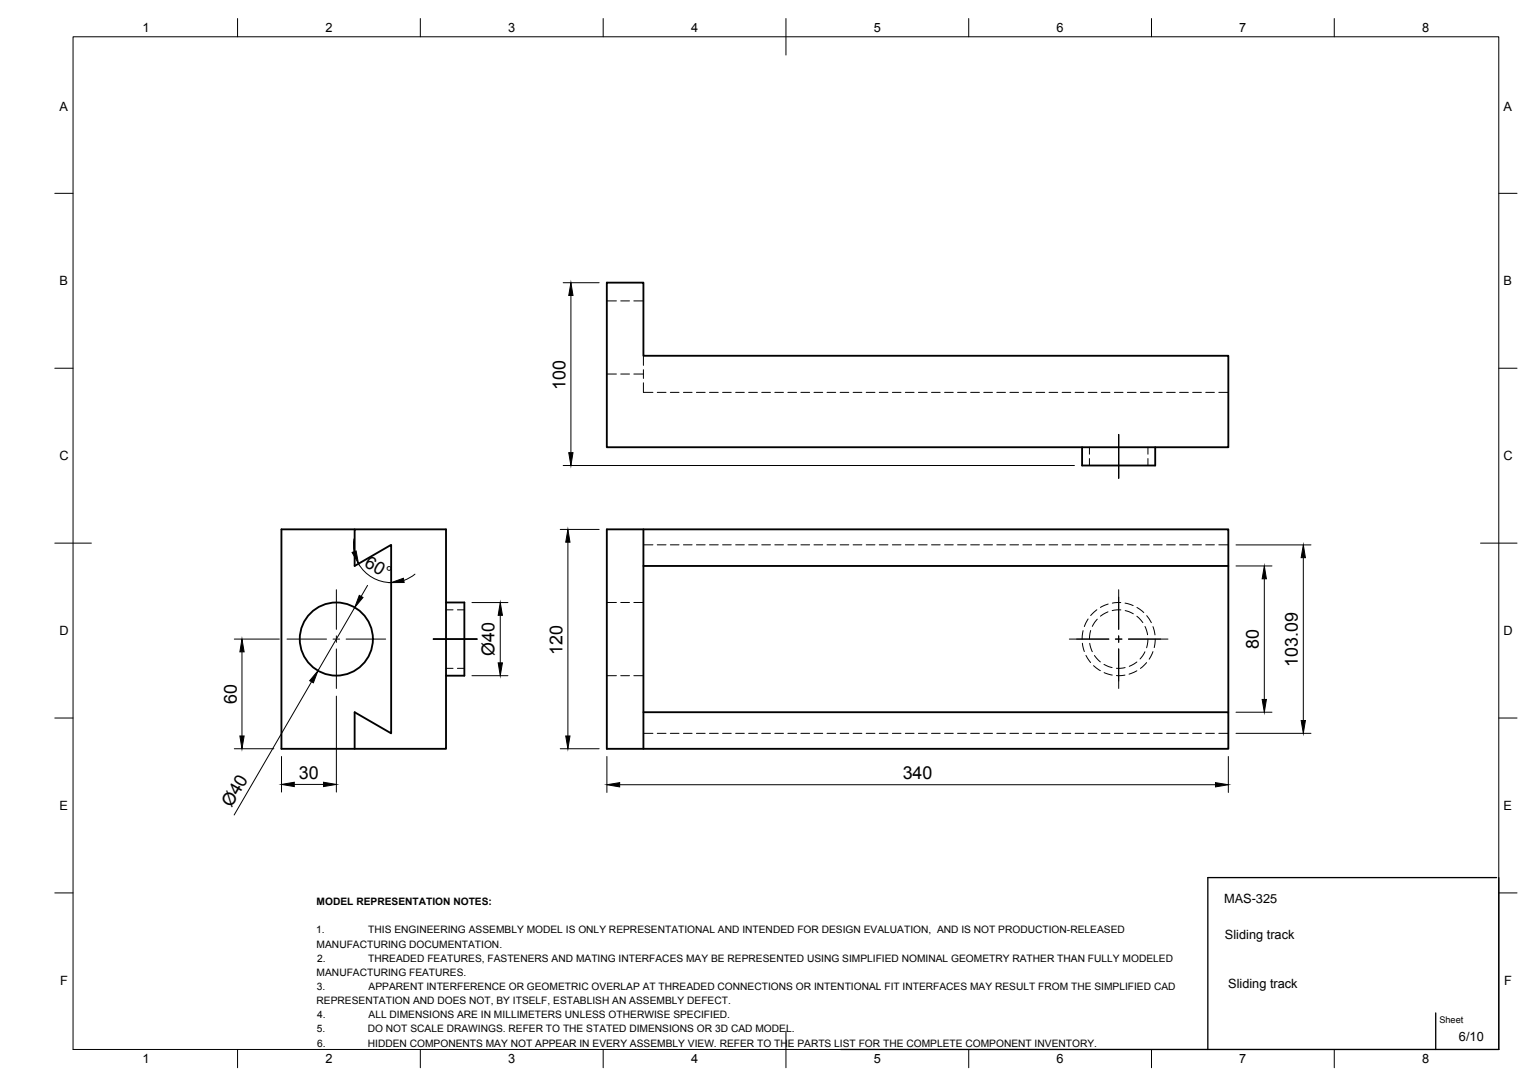
ISO-10303-21;
HEADER;
FILE_DESCRIPTION (('STEP AP214'),
    '1' );
FILE_NAME ('Sliding track.step',
    '2026-10-08T01:23:29',
    ( '' ),
    ( '' ),
    'SwSTEP 2.0',
    'SolidWorks 2025',
    '' );
FILE_SCHEMA (( 'AUTOMOTIVE_DESIGN' ));
ENDSEC;

DATA;
#68=ORIENTED_EDGE ( 'NONE', *, *, #41329, .T. ) ;
#133=LINE ( 'NONE', #35615, #5709 ) ;
#139=EDGE_LOOP ( 'NONE', ( #49981, #10287, #23201, #19361 ) ) ;
#158=DIRECTION ( 'NONE',  ( 0.000000000000000000, 0.000000000000000000, 1.000000000000000000 ) ) ;
#254=CARTESIAN_POINT ( 'NONE',  ( 1.959434878635765131E-15, -63.50000000000000000, 16.00000000000000000 ) ) ;
#289=VECTOR ( 'NONE', #42767, 1000.000000000000000 ) ;
#296=ORIENTED_EDGE ( 'NONE', *, *, #7021, .F. ) ;
#314=CARTESIAN_POINT ( 'NONE',  ( 60.00000000000000000, -113.5000000000000000, 60.00000000000000711 ) ) ;
#367=ADVANCED_FACE ( 'NONE', ( #12542 ), #28557, .F. ) ;
#505=VECTOR ( 'NONE', #2539, 1000.000000000000000 ) ;
#580=DIRECTION ( 'NONE',  ( 0.000000000000000000, 0.000000000000000000, 1.000000000000000000 ) ) ;
#689=AXIS2_PLACEMENT_3D ( 'NONE', #43278, #30663, #18596 ) ;
#692=CARTESIAN_POINT ( 'NONE',  ( 60.00000000000000000, -113.5000000000000000, 60.00000000000000711 ) ) ;
#701=VECTOR ( 'NONE', #47280, 1000.000000000000000 ) ;
#766=ORIENTED_EDGE ( 'NONE', *, *, #47209, .F. ) ;
#828=CARTESIAN_POINT ( 'NONE',  ( -260.0000000000000000, -113.5000000000000000, -40.00000000000001421 ) ) ;
#915=VECTOR ( 'NONE', #37349, 1000.000000000000000 ) ;
#918=FACE_OUTER_BOUND ( 'NONE', #42235, .T. ) ;
#921=EDGE_CURVE ( 'NONE', #5941, #31777, #13986, .T. ) ;
#924=CARTESIAN_POINT ( 'NONE',  ( -260.0000000000000000, -113.5000000000000142, 60.00000000000001421 ) ) ;
#941=CARTESIAN_POINT ( 'NONE',  ( 0.000000000000000000, -53.50000000000000000, 0.000000000000000000 ) ) ;
#1043=PRODUCT_DEFINITION ( 'UNKNOWN', '', #41839, #39510 ) ;
#1058=AXIS2_PLACEMENT_3D ( 'NONE', #5694, #20664, #36698 ) ;
#1110=DIRECTION ( 'NONE',  ( 0.000000000000000000, 0.000000000000000000, -1.000000000000000000 ) ) ;
#1120=CARTESIAN_POINT ( 'NONE',  ( -280.0000000000000000, -63.50000000000000000, 60.00000000000000711 ) ) ;
#1155=DIRECTION ( 'NONE',  ( -0.000000000000000000, 1.156482317317871232E-16, 1.000000000000000000 ) ) ;
#1226=CARTESIAN_POINT ( 'NONE',  ( -260.0000000000000000, -113.5000000000000142, -60.00000000000001421 ) ) ;
#1229=FACE_BOUND ( 'NONE', #16915, .T. ) ;
#1237=ORIENTED_EDGE ( 'NONE', *, *, #23580, .T. ) ;
#1312=ORIENTED_EDGE ( 'NONE', *, *, #8264, .T. ) ;
#1383=CYLINDRICAL_SURFACE ( 'NONE', #44480, 20.00000000000000000 ) ;
#1444=DIRECTION ( 'NONE',  ( 1.000000000000000000, -0.000000000000000000, 0.000000000000000000 ) ) ;
#1544=LINE ( 'NONE', #13627, #43335 ) ;
#1696=CARTESIAN_POINT ( 'NONE',  ( 0.000000000000000000, -53.50000000000000000, 0.000000000000000000 ) ) ;
#1848=FACE_OUTER_BOUND ( 'NONE', #42521, .T. ) ;
#2052=DIRECTION ( 'NONE',  ( -0.000000000000000000, -1.000000000000000000, -0.000000000000000000 ) ) ;
#2064=VERTEX_POINT ( 'NONE', #8952 ) ;
#2160=ORIENTED_EDGE ( 'NONE', *, *, #11113, .T. ) ;
#2332=CARTESIAN_POINT ( 'NONE',  ( 0.000000000000000000, -53.50000000000000000, -16.00000000000000000 ) ) ;
#2380=( GEOMETRIC_REPRESENTATION_CONTEXT ( 3 ) GLOBAL_UNCERTAINTY_ASSIGNED_CONTEXT ( ( #14323 ) ) GLOBAL_UNIT_ASSIGNED_CONTEXT ( ( #38381, #17900, #46534 ) ) REPRESENTATION_CONTEXT ( 'NONE', 'WORKASPACE' ) );
#2539=DIRECTION ( 'NONE',  ( 0.000000000000000000, 0.000000000000000000, -1.000000000000000000 ) ) ;
#2933=VERTEX_POINT ( 'NONE', #36944 ) ;
#3150=EDGE_LOOP ( 'NONE', ( #32702, #7727, #10320, #4760 ) ) ;
#3183=VERTEX_POINT ( 'NONE', #36286 ) ;
#3288=CARTESIAN_POINT ( 'NONE',  ( 60.00000000000001421, -93.32050807568917605, -51.65063509461091940 ) ) ;
#3373=CARTESIAN_POINT ( 'NONE',  ( -365.0160704661291788, -113.5000000000000142, 39.99999999999998579 ) ) ;
#3714=CARTESIAN_POINT ( 'NONE',  ( 0.000000000000000000, 0.000000000000000000, 0.000000000000000000 ) ) ;
#3743=CARTESIAN_POINT ( 'NONE',  ( 0.000000000000000000, -53.50000000000000000, -20.00000000000000000 ) ) ;
#3821=ADVANCED_FACE ( 'NONE', ( #10963 ), #22552, .F. ) ;
#4009=DIRECTION ( 'NONE',  ( 0.000000000000000000, 0.000000000000000000, -1.000000000000000000 ) ) ;
#4143=PLANE ( 'NONE',  #7249 ) ;
#4221=EDGE_LOOP ( 'NONE', ( #16679, #9617, #36250, #32450 ) ) ;
#4245=AXIS2_PLACEMENT_3D ( 'NONE', #17795, #25672, #21740 ) ;
#4287=ORIENTED_EDGE ( 'NONE', *, *, #39827, .F. ) ;
#4303=CARTESIAN_POINT ( 'NONE',  ( 60.00000000000000000, -113.5000000000000142, 39.99999999999998579 ) ) ;
#4341=DIRECTION ( 'NONE',  ( 1.000000000000000000, -0.000000000000000000, -0.000000000000000000 ) ) ;
#4533=ORIENTED_EDGE ( 'NONE', *, *, #35436, .F. ) ;
#4760=ORIENTED_EDGE ( 'NONE', *, *, #22770, .F. ) ;
#4818=EDGE_CURVE ( 'NONE', #34369, #9644, #1544, .T. ) ;
#4962=ORIENTED_EDGE ( 'NONE', *, *, #38155, .F. ) ;
#5036=PLANE ( 'NONE',  #27015 ) ;
#5054=CARTESIAN_POINT ( 'NONE',  ( -280.0000000000000000, -123.5000000000000284, 6.938893903907228378E-15 ) ) ;
#5135=CARTESIAN_POINT ( 'NONE',  ( -260.0000000000000000, -93.50000000000001421, -51.54700538379269403 ) ) ;
#5155=EDGE_LOOP ( 'NONE', ( #28531, #14817, #44995, #43158 ) ) ;
#5277=( LENGTH_UNIT ( ) NAMED_UNIT ( * ) SI_UNIT ( .MILLI., .METRE. ) );
#5485=CIRCLE ( 'NONE', #16387, 20.00000000000000000 ) ;
#5659=CARTESIAN_POINT ( 'NONE',  ( 0.000000000000000000, -53.50000000000000000, 0.000000000000000000 ) ) ;
#5694=CARTESIAN_POINT ( 'NONE',  ( -260.0000000000000000, -123.5000000000000284, 6.938893903907228378E-15 ) ) ;
#5709=VECTOR ( 'NONE', #4341, 1000.000000000000000 ) ;
#5716=AXIS2_PLACEMENT_3D ( 'NONE', #32335, #16600, #17116 ) ;
#5890=CARTESIAN_POINT ( 'NONE',  ( 60.00000000000001421, -93.50000000000002842, -4.038388177301730527E-15 ) ) ;
#5900=LINE ( 'NONE', #7110, #8981 ) ;
#5914=LINE ( 'NONE', #21928, #31488 ) ;
#5941=VERTEX_POINT ( 'NONE', #42846 ) ;
#5959=EDGE_CURVE ( 'NONE', #10174, #9490, #30762, .T. ) ;
#5969=CARTESIAN_POINT ( 'NONE',  ( 60.00000000000000000, -63.50000000000000000, 60.00000000000000711 ) ) ;
#6120=CARTESIAN_POINT ( 'NONE',  ( -260.0000000000000000, -63.50000000000000000, 60.00000000000000711 ) ) ;
#6144=LINE ( 'NONE', #5890, #42526 ) ;
#6277=SHAPE_REPRESENTATION ( 'Sliding track', ( #31742 ), #2380 ) ;
#6290=ORIENTED_EDGE ( 'NONE', *, *, #9346, .F. ) ;
#6361=VECTOR ( 'NONE', #14012, 1000.000000000000000 ) ;
#6417=ORIENTED_EDGE ( 'NONE', *, *, #31098, .F. ) ;
#6488=DIRECTION ( 'NONE',  ( -0.000000000000000000, -0.000000000000000000, 1.000000000000000000 ) ) ;
#6578=VERTEX_POINT ( 'NONE', #25099 ) ;
#6592=COLOUR_RGB ( '', 0.66274510, 0.83137255, 0.94901961) ;
#6676=ORIENTED_EDGE ( 'NONE', *, *, #24658, .F. ) ;
#6827=LINE ( 'NONE', #38616, #40155 ) ;
#7021=EDGE_CURVE ( 'NONE', #31777, #5941, #21156, .T. ) ;
#7110=CARTESIAN_POINT ( 'NONE',  ( -260.0000000000000000, -113.5000000000000000, 60.00000000000000711 ) ) ;
#7144=FACE_OUTER_BOUND ( 'NONE', #5155, .T. ) ;
#7249=AXIS2_PLACEMENT_3D ( 'NONE', #27770, #48016, #12001 ) ;
#7586=CARTESIAN_POINT ( 'NONE',  ( 0.000000000000000000, -53.50000000000000000, 0.000000000000000000 ) ) ;
#7588=ORIENTED_EDGE ( 'NONE', *, *, #45633, .T. ) ;
#7724=DIRECTION ( 'NONE',  ( -1.000000000000000000, -0.000000000000000000, -0.000000000000000000 ) ) ;
#7727=ORIENTED_EDGE ( 'NONE', *, *, #17837, .T. ) ;
#7816=DIRECTION ( 'NONE',  ( 0.000000000000000000, -1.387778780781445182E-16, 1.000000000000000000 ) ) ;
#7906=CARTESIAN_POINT ( 'NONE',  ( -280.0000000000000000, -153.5000000000000284, 60.00000000000002132 ) ) ;
#7930=DIRECTION ( 'NONE',  ( 0.000000000000000000, -0.5000000000000054401, 0.8660254037844354880 ) ) ;
#7931=CYLINDRICAL_SURFACE ( 'NONE', #8788, 20.00000000000000000 ) ;
#8057=ORIENTED_EDGE ( 'NONE', *, *, #41299, .T. ) ;
#8150=VECTOR ( 'NONE', #19445, 1000.000000000000000 ) ;
#8192=AXIS2_PLACEMENT_3D ( 'NONE', #31683, #8795, #28250 ) ;
#8264=EDGE_CURVE ( 'NONE', #24091, #21356, #11704, .T. ) ;
#8377=DIRECTION ( 'NONE',  ( 0.000000000000000000, -1.000000000000000000, -1.387778780781445182E-16 ) ) ;
#8438=DIRECTION ( 'NONE',  ( 1.000000000000000000, 0.000000000000000000, 0.000000000000000000 ) ) ;
#8570=EDGE_CURVE ( 'NONE', #5941, #2933, #22031, .T. ) ;
#8658=ORIENTED_EDGE ( 'NONE', *, *, #24658, .T. ) ;
#8755=FACE_OUTER_BOUND ( 'NONE', #36638, .T. ) ;
#8788=AXIS2_PLACEMENT_3D ( 'NONE', #39228, #35526, #4009 ) ;
#8795=DIRECTION ( 'NONE',  ( 0.000000000000000000, 1.000000000000000000, -1.156482317317871232E-16 ) ) ;
#8952=CARTESIAN_POINT ( 'NONE',  ( -280.0000000000000000, -123.5000000000000284, 20.00000000000002487 ) ) ;
#8981=VECTOR ( 'NONE', #29780, 1000.000000000000000 ) ;
#8998=CARTESIAN_POINT ( 'NONE',  ( 0.000000000000000000, -53.50000000000000000, 0.000000000000000000 ) ) ;
#9039=VECTOR ( 'NONE', #12513, 1000.000000000000000 ) ;
#9046=ORIENTED_EDGE ( 'NONE', *, *, #22833, .F. ) ;
#9346=EDGE_CURVE ( 'NONE', #27143, #6578, #34536, .T. ) ;
#9417=CARTESIAN_POINT ( 'NONE',  ( 60.00000000000000000, -63.50000000000000000, -60.00000000000000711 ) ) ;
#9490=VERTEX_POINT ( 'NONE', #19800 ) ;
#9582=EDGE_CURVE ( 'NONE', #42659, #33404, #48460, .T. ) ;
#9613=VERTEX_POINT ( 'NONE', #30031 ) ;
#9617=ORIENTED_EDGE ( 'NONE', *, *, #24688, .F. ) ;
#9644=VERTEX_POINT ( 'NONE', #41860 ) ;
#9646=ORIENTED_EDGE ( 'NONE', *, *, #9346, .T. ) ;
#9668=EDGE_LOOP ( 'NONE', ( #6676, #40421, #2160, #4533 ) ) ;
#9876=DIRECTION ( 'NONE',  ( 0.000000000000000000, -0.5000000000000054401, -0.8660254037844354880 ) ) ;
#9976=ORIENTED_EDGE ( 'NONE', *, *, #50429, .T. ) ;
#9985=DIRECTION ( 'NONE',  ( 0.000000000000000000, 1.000000000000000000, 0.000000000000000000 ) ) ;
#10078=ORIENTED_EDGE ( 'NONE', *, *, #34010, .T. ) ;
#10160=LINE ( 'NONE', #5969, #505 ) ;
#10174=VERTEX_POINT ( 'NONE', #22607 ) ;
#10179=DIRECTION ( 'NONE',  ( 0.000000000000000000, 1.000000000000000000, -1.156482317317871232E-16 ) ) ;
#10287=ORIENTED_EDGE ( 'NONE', *, *, #22770, .T. ) ;
#10306=FACE_OUTER_BOUND ( 'NONE', #47351, .T. ) ;
#10320=ORIENTED_EDGE ( 'NONE', *, *, #11231, .F. ) ;
#10355=DIRECTION ( 'NONE',  ( 0.000000000000000000, 0.000000000000000000, 1.000000000000000000 ) ) ;
#10409=FACE_OUTER_BOUND ( 'NONE', #3150, .T. ) ;
#10413=PLANE ( 'NONE',  #4245 ) ;
#10467=ADVANCED_FACE ( 'NONE', ( #10306 ), #34992, .F. ) ;
#10473=VECTOR ( 'NONE', #42135, 1000.000000000000227 ) ;
#10502=EDGE_LOOP ( 'NONE', ( #13287, #24330, #25751, #42278 ) ) ;
#10559=DIRECTION ( 'NONE',  ( 0.000000000000000000, -1.000000000000000000, -0.000000000000000000 ) ) ;
#10963=FACE_OUTER_BOUND ( 'NONE', #42153, .T. ) ;
#10972=CARTESIAN_POINT ( 'NONE',  ( 1.959434878635765131E-15, -53.50000000000000000, 16.00000000000000000 ) ) ;
#11049=ADVANCED_FACE ( 'NONE', ( #48315 ), #23866, .F. ) ;
#11113=EDGE_CURVE ( 'NONE', #11286, #13263, #25844, .T. ) ;
#11199=CARTESIAN_POINT ( 'NONE',  ( -280.0000000000000000, -63.50000000000000000, -60.00000000000000711 ) ) ;
#11231=EDGE_CURVE ( 'NONE', #24601, #38717, #6827, .T. ) ;
#11286=VERTEX_POINT ( 'NONE', #42292 ) ;
#11438=CARTESIAN_POINT ( 'NONE',  ( -260.0000000000000000, -123.5000000000000284, 6.938893903907228378E-15 ) ) ;
#11704=LINE ( 'NONE', #29226, #23658 ) ;
#11917=DIRECTION ( 'NONE',  ( -1.000000000000000000, -0.000000000000000000, -0.000000000000000000 ) ) ;
#11931=CIRCLE ( 'NONE', #28734, 16.00000000000000000 ) ;
#12001=DIRECTION ( 'NONE',  ( -1.000000000000000000, 0.000000000000000000, 0.000000000000000000 ) ) ;
#12093=ADVANCED_FACE ( 'NONE', ( #38234 ), #25898, .F. ) ;
#12437=CARTESIAN_POINT ( 'NONE',  ( -113.4314575050762102, -123.5000000000000284, -20.00000000000001066 ) ) ;
#12513=DIRECTION ( 'NONE',  ( 0.000000000000000000, 1.156482317317871232E-16, 1.000000000000000000 ) ) ;
#12542=FACE_OUTER_BOUND ( 'NONE', #31048, .T. ) ;
#12554=APPLICATION_CONTEXT ( 'automotive_design' ) ;
#12556=VERTEX_POINT ( 'NONE', #22090 ) ;
#12562=CARTESIAN_POINT ( 'NONE',  ( -260.0000000000000000, -63.50000000000000000, 60.00000000000000711 ) ) ;
#12734=PLANE ( 'NONE',  #21577 ) ;
#12752=LINE ( 'NONE', #692, #9039 ) ;
#12810=DIRECTION ( 'NONE',  ( 1.000000000000000000, -0.000000000000000000, -0.000000000000000000 ) ) ;
#12886=CARTESIAN_POINT ( 'NONE',  ( 60.00000000000000000, -113.5000000000000000, 60.00000000000000711 ) ) ;
#12897=CIRCLE ( 'NONE', #14566, 20.00000000000000000 ) ;
#12988=ORIENTED_EDGE ( 'NONE', *, *, #50875, .T. ) ;
#13130=CARTESIAN_POINT ( 'NONE',  ( 2.449293598294706513E-15, -53.50000000000000000, 20.00000000000000000 ) ) ;
#13263=VERTEX_POINT ( 'NONE', #47677 ) ;
#13287=ORIENTED_EDGE ( 'NONE', *, *, #22833, .T. ) ;
#13294=STYLED_ITEM ( 'NONE', ( #19467 ), #36319 ) ;
#13351=LINE ( 'NONE', #12562, #26755 ) ;
#13361=LINE ( 'NONE', #9417, #22140 ) ;
#13426=ADVANCED_FACE ( 'NONE', ( #25549 ), #1383, .T. ) ;
#13580=VECTOR ( 'NONE', #30645, 1000.000000000000000 ) ;
#13627=CARTESIAN_POINT ( 'NONE',  ( -365.0160704661291788, -93.50000000000001421, -51.54700538379269403 ) ) ;
#13986=CIRCLE ( 'NONE', #28221, 16.00000000000000000 ) ;
#14012=DIRECTION ( 'NONE',  ( 0.000000000000000000, 1.346129392433909288E-16, -1.000000000000000000 ) ) ;
#14050=FACE_OUTER_BOUND ( 'NONE', #14288, .T. ) ;
#14257=DIRECTION ( 'NONE',  ( 0.000000000000000000, 0.000000000000000000, -1.000000000000000000 ) ) ;
#14260=EDGE_CURVE ( 'NONE', #3183, #2064, #28837, .T. ) ;
#14281=PRODUCT ( 'Sliding track', 'Sliding track', '', ( #16277 ) ) ;
#14288=EDGE_LOOP ( 'NONE', ( #33198, #8658 ) ) ;
#14323=UNCERTAINTY_MEASURE_WITH_UNIT (LENGTH_MEASURE( 1.000000000000000082E-05 ), #38381, 'distance_accuracy_value', 'NONE');
#14350=DIRECTION ( 'NONE',  ( -1.000000000000000000, 0.000000000000000000, 0.000000000000000000 ) ) ;
#14505=ORIENTED_EDGE ( 'NONE', *, *, #24103, .T. ) ;
#14566=AXIS2_PLACEMENT_3D ( 'NONE', #941, #44835, #158 ) ;
#14620=LINE ( 'NONE', #43240, #15107 ) ;
#14709=VERTEX_POINT ( 'NONE', #1120 ) ;
#14733=ORIENTED_EDGE ( 'NONE', *, *, #8570, .T. ) ;
#14793=ORIENTED_EDGE ( 'NONE', *, *, #36819, .F. ) ;
#14817=ORIENTED_EDGE ( 'NONE', *, *, #34010, .F. ) ;
#14833=ORIENTED_EDGE ( 'NONE', *, *, #23580, .F. ) ;
#14852=ORIENTED_EDGE ( 'NONE', *, *, #45633, .F. ) ;
#14894=ORIENTED_EDGE ( 'NONE', *, *, #11113, .F. ) ;
#14982=ADVANCED_FACE ( 'NONE', ( #19479 ), #47622, .F. ) ;
#15085=CARTESIAN_POINT ( 'NONE',  ( 60.00000000000001421, -93.32050807568917605, 51.65063509461090518 ) ) ;
#15107=VECTOR ( 'NONE', #6488, 1000.000000000000000 ) ;
#15128=LINE ( 'NONE', #3288, #44777 ) ;
#15409=ORIENTED_EDGE ( 'NONE', *, *, #50358, .F. ) ;
#15518=ORIENTED_EDGE ( 'NONE', *, *, #22092, .F. ) ;
#15577=FACE_OUTER_BOUND ( 'NONE', #9668, .T. ) ;
#15615=CARTESIAN_POINT ( 'NONE',  ( 60.00000000000000000, -113.5000000000000000, -40.00000000000001421 ) ) ;
#15811=SURFACE_STYLE_USAGE ( .BOTH. , #44690 ) ;
#15901=DIRECTION ( 'NONE',  ( 0.000000000000000000, 0.8660254037844354880, -0.5000000000000054401 ) ) ;
#16138=VECTOR ( 'NONE', #2052, 1000.000000000000000 ) ;
#16277=PRODUCT_CONTEXT ( 'NONE', #18627, 'mechanical' ) ;
#16387=AXIS2_PLACEMENT_3D ( 'NONE', #5659, #34276, #10355 ) ;
#16443=DIRECTION ( 'NONE',  ( 1.000000000000000000, 0.000000000000000000, 0.000000000000000000 ) ) ;
#16600=DIRECTION ( 'NONE',  ( 0.000000000000000000, 1.000000000000000000, 0.000000000000000000 ) ) ;
#16620=ORIENTED_EDGE ( 'NONE', *, *, #45146, .T. ) ;
#16651=ORIENTED_EDGE ( 'NONE', *, *, #51252, .F. ) ;
#16672=CARTESIAN_POINT ( 'NONE',  ( -113.4314575050762102, -123.5000000000000284, 6.938893903907228378E-15 ) ) ;
#16679=ORIENTED_EDGE ( 'NONE', *, *, #37566, .T. ) ;
#16768=CARTESIAN_POINT ( 'NONE',  ( -260.0000000000000000, -63.50000000000000000, -60.00000000000000711 ) ) ;
#16913=VECTOR ( 'NONE', #28035, 1000.000000000000227 ) ;
#16915=EDGE_LOOP ( 'NONE', ( #21760, #45758 ) ) ;
#16955=DIRECTION ( 'NONE',  ( 0.000000000000000000, -0.000000000000000000, 1.000000000000000000 ) ) ;
#17084=ORIENTED_EDGE ( 'NONE', *, *, #50875, .F. ) ;
#17116=DIRECTION ( 'NONE',  ( 0.000000000000000000, 0.000000000000000000, -1.000000000000000000 ) ) ;
#17119=AXIS2_PLACEMENT_3D ( 'NONE', #7906, #47098, #35503 ) ;
#17237=VECTOR ( 'NONE', #41537, 1000.000000000000000 ) ;
#17415=VECTOR ( 'NONE', #22241, 1000.000000000000000 ) ;
#17486=CARTESIAN_POINT ( 'NONE',  ( 0.000000000000000000, -53.50000000000000000, 0.000000000000000000 ) ) ;
#17735=DIRECTION ( 'NONE',  ( 0.000000000000000000, 1.000000000000000000, 0.000000000000000000 ) ) ;
#17795=CARTESIAN_POINT ( 'NONE',  ( -280.0000000000000000, 0.000000000000000000, 0.000000000000000000 ) ) ;
#17837=EDGE_CURVE ( 'NONE', #6578, #38717, #10160, .T. ) ;
#17900=( NAMED_UNIT ( * ) PLANE_ANGLE_UNIT ( ) SI_UNIT ( $, .RADIAN. ) );
#17909=CIRCLE ( 'NONE', #18725, 20.00000000000001776 ) ;
#17970=ADVANCED_FACE ( 'NONE', ( #918 ), #12734, .T. ) ;
#18125=LINE ( 'NONE', #34150, #35992 ) ;
#18344=PLANE ( 'NONE',  #33366 ) ;
#18383=DIRECTION ( 'NONE',  ( 0.000000000000000000, 0.000000000000000000, 1.000000000000000000 ) ) ;
#18596=DIRECTION ( 'NONE',  ( 0.000000000000000000, 0.000000000000000000, -1.000000000000000000 ) ) ;
#18602=DIRECTION ( 'NONE',  ( 0.000000000000000000, 1.000000000000000000, 0.000000000000000000 ) ) ;
#18627=APPLICATION_CONTEXT ( 'automotive_design' ) ;
#18725=AXIS2_PLACEMENT_3D ( 'NONE', #5054, #37355, #28677 ) ;
#18799=DIRECTION ( 'NONE',  ( 0.000000000000000000, 0.000000000000000000, 1.000000000000000000 ) ) ;
#18917=DIRECTION ( 'NONE',  ( -1.000000000000000000, -0.000000000000000000, -0.000000000000000000 ) ) ;
#19028=CARTESIAN_POINT ( 'NONE',  ( 1.959434878635765131E-15, -53.50000000000000000, 16.00000000000000000 ) ) ;
#19073=VECTOR ( 'NONE', #43014, 1000.000000000000000 ) ;
#19337=ORIENTED_EDGE ( 'NONE', *, *, #48870, .F. ) ;
#19347=CARTESIAN_POINT ( 'NONE',  ( 60.00000000000000000, -63.50000000000000000, -60.00000000000000711 ) ) ;
#19361=ORIENTED_EDGE ( 'NONE', *, *, #5959, .T. ) ;
#19369=EDGE_CURVE ( 'NONE', #9644, #9613, #6144, .T. ) ;
#19445=DIRECTION ( 'NONE',  ( -0.000000000000000000, -0.000000000000000000, 1.000000000000000000 ) ) ;
#19467=PRESENTATION_STYLE_ASSIGNMENT (( #15811 ) ) ;
#19479=FACE_OUTER_BOUND ( 'NONE', #4221, .T. ) ;
#19650=VERTEX_POINT ( 'NONE', #828 ) ;
#19800=CARTESIAN_POINT ( 'NONE',  ( -280.0000000000000000, -153.5000000000000284, 60.00000000000002132 ) ) ;
#19930=VECTOR ( 'NONE', #48891, 1000.000000000000000 ) ;
#20123=EDGE_LOOP ( 'NONE', ( #39254, #296 ) ) ;
#20217=SHAPE_DEFINITION_REPRESENTATION ( #41509, #6277 ) ;
#20551=ORIENTED_EDGE ( 'NONE', *, *, #38155, .T. ) ;
#20559=EDGE_LOOP ( 'NONE', ( #7588, #27735, #14505, #68 ) ) ;
#20664=DIRECTION ( 'NONE',  ( 1.000000000000000000, 0.000000000000000000, 0.000000000000000000 ) ) ;
#20674=CARTESIAN_POINT ( 'NONE',  ( -260.0000000000000000, -63.50000000000000000, 60.00000000000000711 ) ) ;
#20871=ADVANCED_FACE ( 'NONE', ( #7144 ), #22664, .F. ) ;
#20927=AXIS2_PLACEMENT_3D ( 'NONE', #34070, #38262, #45920 ) ;
#21051=FACE_BOUND ( 'NONE', #26798, .T. ) ;
#21156=CIRCLE ( 'NONE', #27854, 16.00000000000000000 ) ;
#21328=CARTESIAN_POINT ( 'NONE',  ( -260.0000000000000000, -113.5000000000000000, 60.00000000000000711 ) ) ;
#21354=CARTESIAN_POINT ( 'NONE',  ( 0.000000000000000000, -53.50000000000000000, 0.000000000000000000 ) ) ;
#21356=VERTEX_POINT ( 'NONE', #32486 ) ;
#21373=EDGE_CURVE ( 'NONE', #49425, #46727, #12752, .T. ) ;
#21397=LINE ( 'NONE', #33498, #44481 ) ;
#21400=AXIS2_PLACEMENT_3D ( 'NONE', #16672, #11917, #31897 ) ;
#21418=VECTOR ( 'NONE', #40158, 1000.000000000000000 ) ;
#21561=( NAMED_UNIT ( * ) SI_UNIT ( $, .STERADIAN. ) SOLID_ANGLE_UNIT ( ) );
#21566=ORIENTED_EDGE ( 'NONE', *, *, #48018, .F. ) ;
#21577=AXIS2_PLACEMENT_3D ( 'NONE', #44552, #1444, #25360 ) ;
#21740=DIRECTION ( 'NONE',  ( 0.000000000000000000, 0.000000000000000000, -1.000000000000000000 ) ) ;
#21760=ORIENTED_EDGE ( 'NONE', *, *, #50429, .F. ) ;
#21774=CARTESIAN_POINT ( 'NONE',  ( 0.000000000000000000, -63.50000000000000000, 0.000000000000000000 ) ) ;
#21858=LINE ( 'NONE', #21328, #915 ) ;
#21928=CARTESIAN_POINT ( 'NONE',  ( -280.0000000000000000, -153.5000000000000284, 60.00000000000002132 ) ) ;
#22031=LINE ( 'NONE', #2332, #16138 ) ;
#22084=CARTESIAN_POINT ( 'NONE',  ( -113.4314575050762102, -123.5000000000000284, 6.938893903907228378E-15 ) ) ;
#22090=CARTESIAN_POINT ( 'NONE',  ( -260.0000000000000000, -93.50000000000002842, 51.54700538379266561 ) ) ;
#22092=EDGE_CURVE ( 'NONE', #9490, #14709, #43671, .T. ) ;
#22096=SHAPE_REPRESENTATION_RELATIONSHIP ( 'NONE' , 'NONE' ,  #6277, #39951 ) ;
#22140=VECTOR ( 'NONE', #8377, 1000.000000000000000 ) ;
#22241=DIRECTION ( 'NONE',  ( 0.000000000000000000, 0.000000000000000000, -1.000000000000000000 ) ) ;
#22314=VERTEX_POINT ( 'NONE', #924 ) ;
#22527=EDGE_LOOP ( 'NONE', ( #33410, #51745, #25450, #33288 ) ) ;
#22552=CYLINDRICAL_SURFACE ( 'NONE', #689, 16.00000000000000000 ) ;
#22553=ORIENTED_EDGE ( 'NONE', *, *, #41299, .F. ) ;
#22607=CARTESIAN_POINT ( 'NONE',  ( -280.0000000000000000, -153.5000000000000284, -59.99999999999999289 ) ) ;
#22664=PLANE ( 'NONE',  #27441 ) ;
#22770=EDGE_CURVE ( 'NONE', #14709, #24601, #50894, .T. ) ;
#22833=EDGE_CURVE ( 'NONE', #3183, #42659, #35062, .T. ) ;
#22869=EDGE_CURVE ( 'NONE', #24091, #49425, #133, .T. ) ;
#22967=LINE ( 'NONE', #19028, #36187 ) ;
#23201=ORIENTED_EDGE ( 'NONE', *, *, #39827, .T. ) ;
#23358=ORIENTED_EDGE ( 'NONE', *, *, #50358, .T. ) ;
#23579=FACE_OUTER_BOUND ( 'NONE', #51758, .T. ) ;
#23580=EDGE_CURVE ( 'NONE', #40297, #47963, #30708, .T. ) ;
#23658=VECTOR ( 'NONE', #23794, 1000.000000000000000 ) ;
#23678=DIRECTION ( 'NONE',  ( 0.000000000000000000, 1.000000000000000000, 1.346129392433909288E-16 ) ) ;
#23794=DIRECTION ( 'NONE',  ( 0.000000000000000000, -1.000000000000000000, 1.541976423090494894E-16 ) ) ;
#23808=LINE ( 'NONE', #11199, #13580 ) ;
#23866=CYLINDRICAL_SURFACE ( 'NONE', #26702, 16.00000000000000000 ) ;
#23929=ORIENTED_EDGE ( 'NONE', *, *, #48870, .T. ) ;
#24091=VERTEX_POINT ( 'NONE', #1226 ) ;
#24103=EDGE_CURVE ( 'NONE', #34369, #19650, #44364, .T. ) ;
#24153=ORIENTED_EDGE ( 'NONE', *, *, #49529, .F. ) ;
#24205=ORIENTED_EDGE ( 'NONE', *, *, #35436, .T. ) ;
#24228=CARTESIAN_POINT ( 'NONE',  ( 60.00000000000000000, -113.5000000000000142, -60.00000000000001421 ) ) ;
#24286=ADVANCED_FACE ( 'NONE', ( #26172, #10409 ), #49853, .F. ) ;
#24330=ORIENTED_EDGE ( 'NONE', *, *, #9582, .T. ) ;
#24375=AXIS2_PLACEMENT_3D ( 'NONE', #27657, #7930, #47647 ) ;
#24377=CARTESIAN_POINT ( 'NONE',  ( -260.0000000000000000, -113.5000000000000000, -40.00000000000001421 ) ) ;
#24566=ORIENTED_EDGE ( 'NONE', *, *, #47209, .T. ) ;
#24601=VERTEX_POINT ( 'NONE', #42410 ) ;
#24658=EDGE_CURVE ( 'NONE', #27596, #33838, #5485, .T. ) ;
#24688=EDGE_CURVE ( 'NONE', #9490, #39530, #5914, .T. ) ;
#24724=CARTESIAN_POINT ( 'NONE',  ( -260.0000000000000000, -113.5000000000000000, 60.00000000000000711 ) ) ;
#24909=VECTOR ( 'NONE', #7724, 1000.000000000000000 ) ;
#25004=DIRECTION ( 'NONE',  ( 0.000000000000000000, 0.000000000000000000, -1.000000000000000000 ) ) ;
#25067=LINE ( 'NONE', #49512, #6361 ) ;
#25099=CARTESIAN_POINT ( 'NONE',  ( 60.00000000000000000, -63.50000000000000000, 60.00000000000000711 ) ) ;
#25102=DIRECTION ( 'NONE',  ( 0.000000000000000000, 1.000000000000000000, 0.000000000000000000 ) ) ;
#25268=LINE ( 'NONE', #29204, #17237 ) ;
#25360=DIRECTION ( 'NONE',  ( 0.000000000000000000, 0.000000000000000000, -1.000000000000000000 ) ) ;
#25394=CARTESIAN_POINT ( 'NONE',  ( -260.0000000000000000, -123.5000000000000284, -20.00000000000001066 ) ) ;
#25416=ORIENTED_EDGE ( 'NONE', *, *, #11231, .T. ) ;
#25446=AXIS2_PLACEMENT_3D ( 'NONE', #16768, #7816, #28037 ) ;
#25450=ORIENTED_EDGE ( 'NONE', *, *, #45146, .F. ) ;
#25549=FACE_OUTER_BOUND ( 'NONE', #29952, .T. ) ;
#25672=DIRECTION ( 'NONE',  ( 1.000000000000000000, 0.000000000000000000, 0.000000000000000000 ) ) ;
#25705=ORIENTED_EDGE ( 'NONE', *, *, #21373, .F. ) ;
#25751=ORIENTED_EDGE ( 'NONE', *, *, #41069, .T. ) ;
#25844=CIRCLE ( 'NONE', #5716, 20.00000000000000000 ) ;
#25898=PLANE ( 'NONE',  #40198 ) ;
#25900=ADVANCED_FACE ( 'NONE', ( #36056 ), #39227, .F. ) ;
#26172=FACE_BOUND ( 'NONE', #46638, .T. ) ;
#26198=DIRECTION ( 'NONE',  ( 0.000000000000000000, 1.156482317317871232E-16, 1.000000000000000000 ) ) ;
#26702=AXIS2_PLACEMENT_3D ( 'NONE', #7586, #32010, #39882 ) ;
#26755=VECTOR ( 'NONE', #12810, 1000.000000000000000 ) ;
#26777=EDGE_CURVE ( 'NONE', #40297, #12556, #48561, .T. ) ;
#26789=DIRECTION ( 'NONE',  ( 1.000000000000000000, -0.000000000000000000, -0.000000000000000000 ) ) ;
#26798=EDGE_LOOP ( 'NONE', ( #9046, #27115 ) ) ;
#26980=CARTESIAN_POINT ( 'NONE',  ( -280.0000000000000000, -153.5000000000000284, -59.99999999999999289 ) ) ;
#27015=AXIS2_PLACEMENT_3D ( 'NONE', #32865, #45748, #25004 ) ;
#27065=CARTESIAN_POINT ( 'NONE',  ( -280.0000000000000000, -153.5000000000000284, 60.00000000000002132 ) ) ;
#27087=CARTESIAN_POINT ( 'NONE',  ( -260.0000000000000000, -153.5000000000000284, 60.00000000000002132 ) ) ;
#27115=ORIENTED_EDGE ( 'NONE', *, *, #45388, .F. ) ;
#27143=VERTEX_POINT ( 'NONE', #314 ) ;
#27374=CARTESIAN_POINT ( 'NONE',  ( -280.0000000000000000, -63.50000000000000000, 60.00000000000000711 ) ) ;
#27441=AXIS2_PLACEMENT_3D ( 'NONE', #42881, #23678, #39199 ) ;
#27449=VERTEX_POINT ( 'NONE', #254 ) ;
#27596=VERTEX_POINT ( 'NONE', #13130 ) ;
#27657=CARTESIAN_POINT ( 'NONE',  ( -365.0160704661291788, -93.50000000000002842, 51.54700538379266561 ) ) ;
#27735=ORIENTED_EDGE ( 'NONE', *, *, #4818, .F. ) ;
#27770=CARTESIAN_POINT ( 'NONE',  ( -260.0000000000000000, -63.50000000000000000, 60.00000000000000711 ) ) ;
#27854=AXIS2_PLACEMENT_3D ( 'NONE', #8998, #40251, #580 ) ;
#28035=DIRECTION ( 'NONE',  ( -0.000000000000000000, 0.8660254037844354880, 0.5000000000000054401 ) ) ;
#28037=DIRECTION ( 'NONE',  ( 0.000000000000000000, -1.000000000000000000, -1.387778780781445182E-16 ) ) ;
#28065=ORIENTED_EDGE ( 'NONE', *, *, #22869, .T. ) ;
#28209=AXIS2_PLACEMENT_3D ( 'NONE', #21774, #18602, #46723 ) ;
#28221=AXIS2_PLACEMENT_3D ( 'NONE', #17486, #25102, #33502 ) ;
#28250=DIRECTION ( 'NONE',  ( 0.000000000000000000, 1.156482317317871232E-16, 1.000000000000000000 ) ) ;
#28330=AXIS2_PLACEMENT_3D ( 'NONE', #11438, #16443, #40322 ) ;
#28390=ADVANCED_FACE ( 'NONE', ( #14050, #33228 ), #49543, .T. ) ;
#28501=AXIS2_PLACEMENT_3D ( 'NONE', #37822, #9985, #18383 ) ;
#28531=ORIENTED_EDGE ( 'NONE', *, *, #19369, .T. ) ;
#28555=CARTESIAN_POINT ( 'NONE',  ( -260.0000000000000000, -93.50000000000002842, 51.54700538379266561 ) ) ;
#28557=PLANE ( 'NONE',  #25446 ) ;
#28677=DIRECTION ( 'NONE',  ( 0.000000000000000000, 0.000000000000000000, 1.000000000000000000 ) ) ;
#28734=AXIS2_PLACEMENT_3D ( 'NONE', #45961, #30668, #46986 ) ;
#28837=LINE ( 'NONE', #32536, #21418 ) ;
#29204=CARTESIAN_POINT ( 'NONE',  ( 2.449293598294706513E-15, -53.50000000000000000, 20.00000000000000000 ) ) ;
#29226=CARTESIAN_POINT ( 'NONE',  ( -260.0000000000000000, -63.50000000000000000, -60.00000000000000711 ) ) ;
#29764=ORIENTED_EDGE ( 'NONE', *, *, #43692, .T. ) ;
#29780=DIRECTION ( 'NONE',  ( 1.000000000000000000, -0.000000000000000000, -0.000000000000000000 ) ) ;
#29834=ORIENTED_EDGE ( 'NONE', *, *, #17837, .F. ) ;
#29952=EDGE_LOOP ( 'NONE', ( #24153, #30154, #24205, #23929 ) ) ;
#30031=CARTESIAN_POINT ( 'NONE',  ( 60.00000000000000000, -93.50000000000002842, 51.54700538379266561 ) ) ;
#30124=ADVANCED_FACE ( 'NONE', ( #15577 ), #7931, .T. ) ;
#30154=ORIENTED_EDGE ( 'NONE', *, *, #41666, .F. ) ;
#30212=DIRECTION ( 'NONE',  ( -0.000000000000000000, -1.000000000000000000, -0.000000000000000000 ) ) ;
#30591=CARTESIAN_POINT ( 'NONE',  ( 60.00000000000000000, -63.50000000000000000, 60.00000000000000711 ) ) ;
#30611=CARTESIAN_POINT ( 'NONE',  ( -280.0000000000000000, -123.5000000000000284, 6.938893903907228378E-15 ) ) ;
#30645=DIRECTION ( 'NONE',  ( 0.000000000000000000, -1.000000000000000000, 1.541976423090494894E-16 ) ) ;
#30663=DIRECTION ( 'NONE',  ( -0.000000000000000000, -1.000000000000000000, -0.000000000000000000 ) ) ;
#30668=DIRECTION ( 'NONE',  ( 0.000000000000000000, 1.000000000000000000, 0.000000000000000000 ) ) ;
#30708=LINE ( 'NONE', #3373, #701 ) ;
#30723=ORIENTED_EDGE ( 'NONE', *, *, #31239, .F. ) ;
#30762=LINE ( 'NONE', #27065, #8150 ) ;
#31048=EDGE_LOOP ( 'NONE', ( #25416, #8057, #50272, #1312, #16651, #4287 ) ) ;
#31098=EDGE_CURVE ( 'NONE', #40297, #22314, #21397, .T. ) ;
#31239=EDGE_CURVE ( 'NONE', #9613, #47963, #35038, .T. ) ;
#31488=VECTOR ( 'NONE', #33231, 1000.000000000000000 ) ;
#31587=VECTOR ( 'NONE', #49584, 1000.000000000000000 ) ;
#31683=CARTESIAN_POINT ( 'NONE',  ( -260.0000000000000000, -113.5000000000000000, 60.00000000000000711 ) ) ;
#31703=ORIENTED_EDGE ( 'NONE', *, *, #26777, .T. ) ;
#31742=AXIS2_PLACEMENT_3D ( 'NONE', #3714, #31843, #8438 ) ;
#31777=VERTEX_POINT ( 'NONE', #10972 ) ;
#31843=DIRECTION ( 'NONE',  ( 0.000000000000000000, 0.000000000000000000, 1.000000000000000000 ) ) ;
#31897=DIRECTION ( 'NONE',  ( 0.000000000000000000, 0.000000000000000000, 1.000000000000000000 ) ) ;
#31940=ORIENTED_EDGE ( 'NONE', *, *, #7021, .T. ) ;
#32010=DIRECTION ( 'NONE',  ( -0.000000000000000000, -1.000000000000000000, -0.000000000000000000 ) ) ;
#32112=CLOSED_SHELL ( 'NONE', ( #11049, #30124, #48443, #51073, #50342, #24286, #367, #34330, #17970, #14982, #38636, #44572, #25900, #20871, #12093, #47851, #28390, #13426, #3821, #10467 ) ) ;
#32335=CARTESIAN_POINT ( 'NONE',  ( 0.000000000000000000, -63.50000000000000000, 0.000000000000000000 ) ) ;
#32380=ORIENTED_EDGE ( 'NONE', *, *, #19369, .F. ) ;
#32410=CIRCLE ( 'NONE', #39119, 20.00000000000001776 ) ;
#32450=ORIENTED_EDGE ( 'NONE', *, *, #51252, .T. ) ;
#32486=CARTESIAN_POINT ( 'NONE',  ( -260.0000000000000000, -153.5000000000000284, -59.99999999999999289 ) ) ;
#32536=CARTESIAN_POINT ( 'NONE',  ( -113.4314575050762102, -123.5000000000000284, 20.00000000000002487 ) ) ;
#32702=ORIENTED_EDGE ( 'NONE', *, *, #36819, .T. ) ;
#32865=CARTESIAN_POINT ( 'NONE',  ( -260.0000000000000000, 0.000000000000000000, 0.000000000000000000 ) ) ;
#32999=ORIENTED_EDGE ( 'NONE', *, *, #9582, .F. ) ;
#33049=ORIENTED_EDGE ( 'NONE', *, *, #21373, .T. ) ;
#33136=VECTOR ( 'NONE', #45485, 1000.000000000000000 ) ;
#33198=ORIENTED_EDGE ( 'NONE', *, *, #41666, .T. ) ;
#33228=FACE_BOUND ( 'NONE', #20123, .T. ) ;
#33231=DIRECTION ( 'NONE',  ( 1.000000000000000000, -0.000000000000000000, -0.000000000000000000 ) ) ;
#33284=EDGE_LOOP ( 'NONE', ( #6417, #1237, #24566, #17084 ) ) ;
#33288=ORIENTED_EDGE ( 'NONE', *, *, #8570, .F. ) ;
#33366=AXIS2_PLACEMENT_3D ( 'NONE', #24724, #10179, #26198 ) ;
#33404=VERTEX_POINT ( 'NONE', #50646 ) ;
#33410=ORIENTED_EDGE ( 'NONE', *, *, #921, .T. ) ;
#33497=VECTOR ( 'NONE', #40380, 1000.000000000000227 ) ;
#33498=CARTESIAN_POINT ( 'NONE',  ( -260.0000000000000000, -113.5000000000000000, 60.00000000000000711 ) ) ;
#33502=DIRECTION ( 'NONE',  ( 0.000000000000000000, 0.000000000000000000, 1.000000000000000000 ) ) ;
#33643=LINE ( 'NONE', #12886, #33136 ) ;
#33648=ORIENTED_EDGE ( 'NONE', *, *, #43692, .F. ) ;
#33838=VERTEX_POINT ( 'NONE', #3743 ) ;
#33908=DIRECTION ( 'NONE',  ( 0.000000000000000000, 0.000000000000000000, 1.000000000000000000 ) ) ;
#33978=ORIENTED_EDGE ( 'NONE', *, *, #24103, .F. ) ;
#34010=EDGE_CURVE ( 'NONE', #12556, #9613, #48635, .T. ) ;
#34070=CARTESIAN_POINT ( 'NONE',  ( -260.0000000000000000, -63.50000000000000000, 60.00000000000000711 ) ) ;
#34150=CARTESIAN_POINT ( 'NONE',  ( 0.000000000000000000, -53.50000000000000000, -20.00000000000000000 ) ) ;
#34158=VECTOR ( 'NONE', #38938, 1000.000000000000000 ) ;
#34276=DIRECTION ( 'NONE',  ( 0.000000000000000000, 1.000000000000000000, 0.000000000000000000 ) ) ;
#34330=ADVANCED_FACE ( 'NONE', ( #44549 ), #47729, .F. ) ;
#34369=VERTEX_POINT ( 'NONE', #5135 ) ;
#34536=LINE ( 'NONE', #30591, #50053 ) ;
#34676=AXIS2_PLACEMENT_3D ( 'NONE', #1696, #17735, #16955 ) ;
#34992=PLANE ( 'NONE',  #51856 ) ;
#35038=LINE ( 'NONE', #15085, #10473 ) ;
#35062=CIRCLE ( 'NONE', #28330, 20.00000000000001776 ) ;
#35171=ORIENTED_EDGE ( 'NONE', *, *, #45388, .T. ) ;
#35314=UNCERTAINTY_MEASURE_WITH_UNIT (LENGTH_MEASURE( 1.000000000000000082E-05 ), #5277, 'distance_accuracy_value', 'NONE');
#35436=EDGE_CURVE ( 'NONE', #33838, #13263, #18125, .T. ) ;
#35503=DIRECTION ( 'NONE',  ( 0.000000000000000000, -0.000000000000000000, 1.000000000000000000 ) ) ;
#35526=DIRECTION ( 'NONE',  ( -0.000000000000000000, -1.000000000000000000, -0.000000000000000000 ) ) ;
#35615=CARTESIAN_POINT ( 'NONE',  ( -260.0000000000000000, -113.5000000000000142, -60.00000000000001421 ) ) ;
#35753=FILL_AREA_STYLE_COLOUR ( '', #6592 ) ;
#35992=VECTOR ( 'NONE', #30212, 1000.000000000000000 ) ;
#36056=FACE_OUTER_BOUND ( 'NONE', #43479, .T. ) ;
#36187=VECTOR ( 'NONE', #51112, 1000.000000000000000 ) ;
#36250=ORIENTED_EDGE ( 'NONE', *, *, #5959, .F. ) ;
#36286=CARTESIAN_POINT ( 'NONE',  ( -260.0000000000000000, -123.5000000000000284, 20.00000000000002487 ) ) ;
#36319=MANIFOLD_SOLID_BREP ( 'Boss-Extrude10', #32112 ) ;
#36462=ORIENTED_EDGE ( 'NONE', *, *, #41329, .F. ) ;
#36517=CARTESIAN_POINT ( 'NONE',  ( -365.0160704661291788, -93.50000000000002842, 51.54700538379266561 ) ) ;
#36638=EDGE_LOOP ( 'NONE', ( #32999, #35171, #51280, #9976 ) ) ;
#36698=DIRECTION ( 'NONE',  ( 0.000000000000000000, 0.000000000000000000, -1.000000000000000000 ) ) ;
#36800=ORIENTED_EDGE ( 'NONE', *, *, #26777, .F. ) ;
#36819=EDGE_CURVE ( 'NONE', #14709, #6578, #13351, .T. ) ;
#36885=CYLINDRICAL_SURFACE ( 'NONE', #21400, 20.00000000000001776 ) ;
#36944=CARTESIAN_POINT ( 'NONE',  ( 0.000000000000000000, -63.50000000000000000, -16.00000000000000000 ) ) ;
#37349=DIRECTION ( 'NONE',  ( -0.000000000000000000, 1.156482317317871232E-16, 1.000000000000000000 ) ) ;
#37355=DIRECTION ( 'NONE',  ( -1.000000000000000000, 0.000000000000000000, 0.000000000000000000 ) ) ;
#37566=EDGE_CURVE ( 'NONE', #21356, #39530, #14620, .T. ) ;
#37792=DIRECTION ( 'NONE',  ( 1.000000000000000000, -0.000000000000000000, -0.000000000000000000 ) ) ;
#37822=CARTESIAN_POINT ( 'NONE',  ( 0.000000000000000000, -63.50000000000000000, 0.000000000000000000 ) ) ;
#38155=EDGE_CURVE ( 'NONE', #27449, #2933, #51225, .T. ) ;
#38234=FACE_OUTER_BOUND ( 'NONE', #20559, .T. ) ;
#38262=DIRECTION ( 'NONE',  ( 0.000000000000000000, -1.000000000000000000, -0.000000000000000000 ) ) ;
#38381=( LENGTH_UNIT ( ) NAMED_UNIT ( * ) SI_UNIT ( .MILLI., .METRE. ) );
#38458=( GEOMETRIC_REPRESENTATION_CONTEXT ( 3 ) GLOBAL_UNCERTAINTY_ASSIGNED_CONTEXT ( ( #35314 ) ) GLOBAL_UNIT_ASSIGNED_CONTEXT ( ( #5277, #41789, #21561 ) ) REPRESENTATION_CONTEXT ( 'NONE', 'WORKASPACE' ) );
#38616=CARTESIAN_POINT ( 'NONE',  ( -260.0000000000000000, -63.50000000000000000, -60.00000000000000711 ) ) ;
#38636=ADVANCED_FACE ( 'NONE', ( #1229, #49347 ), #10413, .F. ) ;
#38693=DIRECTION ( 'NONE',  ( -0.000000000000000000, -1.346129392433909288E-16, 1.000000000000000000 ) ) ;
#38717=VERTEX_POINT ( 'NONE', #19347 ) ;
#38938=DIRECTION ( 'NONE',  ( -0.000000000000000000, 1.000000000000000000, -1.541976423090494894E-16 ) ) ;
#39006=CIRCLE ( 'NONE', #28209, 20.00000000000000000 ) ;
#39100=EDGE_CURVE ( 'NONE', #31777, #27449, #22967, .T. ) ;
#39119=AXIS2_PLACEMENT_3D ( 'NONE', #30611, #14350, #18799 ) ;
#39199=DIRECTION ( 'NONE',  ( 0.000000000000000000, -1.346129392433909288E-16, 1.000000000000000000 ) ) ;
#39227=PLANE ( 'NONE',  #24375 ) ;
#39228=CARTESIAN_POINT ( 'NONE',  ( 0.000000000000000000, -53.50000000000000000, 0.000000000000000000 ) ) ;
#39254=ORIENTED_EDGE ( 'NONE', *, *, #921, .F. ) ;
#39510=PRODUCT_DEFINITION_CONTEXT ( 'detailed design', #12554, 'design' ) ;
#39530=VERTEX_POINT ( 'NONE', #27087 ) ;
#39827=EDGE_CURVE ( 'NONE', #24601, #10174, #23808, .T. ) ;
#39882=DIRECTION ( 'NONE',  ( 0.000000000000000000, 0.000000000000000000, -1.000000000000000000 ) ) ;
#39939=AXIS2_PLACEMENT_3D ( 'NONE', #22084, #18917, #33908 ) ;
#39951=ADVANCED_BREP_SHAPE_REPRESENTATION ( '', ( #36319, #31742 ), #2380 ) ;
#40155=VECTOR ( 'NONE', #26789, 1000.000000000000000 ) ;
#40158=DIRECTION ( 'NONE',  ( -1.000000000000000000, -0.000000000000000000, -0.000000000000000000 ) ) ;
#40198=AXIS2_PLACEMENT_3D ( 'NONE', #42438, #9876, #41925 ) ;
#40251=DIRECTION ( 'NONE',  ( 0.000000000000000000, 1.000000000000000000, 0.000000000000000000 ) ) ;
#40297=VERTEX_POINT ( 'NONE', #47925 ) ;
#40322=DIRECTION ( 'NONE',  ( 0.000000000000000000, 0.000000000000000000, -1.000000000000000000 ) ) ;
#40380=DIRECTION ( 'NONE',  ( 0.000000000000000000, -0.8660254037844354880, 0.5000000000000054401 ) ) ;
#40421=ORIENTED_EDGE ( 'NONE', *, *, #49529, .T. ) ;
#40457=ORIENTED_EDGE ( 'NONE', *, *, #37566, .F. ) ;
#41069=EDGE_CURVE ( 'NONE', #33404, #2064, #17909, .T. ) ;
#41084=MECHANICAL_DESIGN_GEOMETRIC_PRESENTATION_REPRESENTATION('',(#13294),#38458);
#41299=EDGE_CURVE ( 'NONE', #38717, #49425, #13361, .T. ) ;
#41329=EDGE_CURVE ( 'NONE', #19650, #46727, #46456, .T. ) ;
#41509=PRODUCT_DEFINITION_SHAPE ( 'NONE', 'NONE',  #1043 ) ;
#41537=DIRECTION ( 'NONE',  ( -0.000000000000000000, -1.000000000000000000, -0.000000000000000000 ) ) ;
#41573=DIRECTION ( 'NONE',  ( -0.000000000000000000, -1.000000000000000000, -0.000000000000000000 ) ) ;
#41666=EDGE_CURVE ( 'NONE', #33838, #27596, #12897, .T. ) ;
#41789=( NAMED_UNIT ( * ) PLANE_ANGLE_UNIT ( ) SI_UNIT ( $, .RADIAN. ) );
#41839=PRODUCT_DEFINITION_FORMATION_WITH_SPECIFIED_SOURCE ( 'ANY', '', #14281, .NOT_KNOWN. ) ;
#41860=CARTESIAN_POINT ( 'NONE',  ( 60.00000000000000000, -93.50000000000001421, -51.54700538379269403 ) ) ;
#41925=DIRECTION ( 'NONE',  ( 0.000000000000000000, 0.8660254037844354880, -0.5000000000000054401 ) ) ;
#42054=FACE_OUTER_BOUND ( 'NONE', #10502, .T. ) ;
#42135=DIRECTION ( 'NONE',  ( 0.000000000000000000, -0.8660254037844354880, -0.5000000000000054401 ) ) ;
#42153=EDGE_LOOP ( 'NONE', ( #51199, #31940, #14733, #4962 ) ) ;
#42235=EDGE_LOOP ( 'NONE', ( #30723, #32380, #14852, #25705, #22553, #29834, #6290, #766 ) ) ;
#42278=ORIENTED_EDGE ( 'NONE', *, *, #14260, .F. ) ;
#42292=CARTESIAN_POINT ( 'NONE',  ( 2.449293598294706513E-15, -63.50000000000000000, 20.00000000000000000 ) ) ;
#42410=CARTESIAN_POINT ( 'NONE',  ( -280.0000000000000000, -63.50000000000000000, -60.00000000000000711 ) ) ;
#42438=CARTESIAN_POINT ( 'NONE',  ( -365.0160704661291788, -113.5000000000000000, -40.00000000000001421 ) ) ;
#42521=EDGE_LOOP ( 'NONE', ( #43482, #29764, #33978, #21566, #36800, #44685, #15409, #40457 ) ) ;
#42526=VECTOR ( 'NONE', #38693, 1000.000000000000000 ) ;
#42659=VERTEX_POINT ( 'NONE', #25394 ) ;
#42767=DIRECTION ( 'NONE',  ( 1.000000000000000000, -0.000000000000000000, -0.000000000000000000 ) ) ;
#42846=CARTESIAN_POINT ( 'NONE',  ( 0.000000000000000000, -53.50000000000000000, -16.00000000000000000 ) ) ;
#42881=CARTESIAN_POINT ( 'NONE',  ( -365.0160704661291788, -93.50000000000001421, -51.54700538379269403 ) ) ;
#42901=EDGE_LOOP ( 'NONE', ( #33049, #36462, #33648, #28065 ) ) ;
#43014=DIRECTION ( 'NONE',  ( 1.000000000000000000, -0.000000000000000000, -0.000000000000000000 ) ) ;
#43158=ORIENTED_EDGE ( 'NONE', *, *, #4818, .T. ) ;
#43240=CARTESIAN_POINT ( 'NONE',  ( -260.0000000000000000, -153.5000000000000284, 60.00000000000002132 ) ) ;
#43245=CARTESIAN_POINT ( 'NONE',  ( -280.0000000000000000, -63.50000000000000000, 60.00000000000000711 ) ) ;
#43278=CARTESIAN_POINT ( 'NONE',  ( 0.000000000000000000, -53.50000000000000000, 0.000000000000000000 ) ) ;
#43335=VECTOR ( 'NONE', #37792, 1000.000000000000000 ) ;
#43479=EDGE_LOOP ( 'NONE', ( #50185, #14833, #31703, #10078 ) ) ;
#43482=ORIENTED_EDGE ( 'NONE', *, *, #8264, .F. ) ;
#43671=LINE ( 'NONE', #27374, #34158 ) ;
#43692=EDGE_CURVE ( 'NONE', #24091, #19650, #21858, .T. ) ;
#43861=CIRCLE ( 'NONE', #1058, 20.00000000000001776 ) ;
#44364=LINE ( 'NONE', #24377, #33497 ) ;
#44480=AXIS2_PLACEMENT_3D ( 'NONE', #21354, #41573, #1110 ) ;
#44481=VECTOR ( 'NONE', #1155, 1000.000000000000000 ) ;
#44549=FACE_OUTER_BOUND ( 'NONE', #42901, .T. ) ;
#44552=CARTESIAN_POINT ( 'NONE',  ( 60.00000000000001421, -63.50000000000000000, 0.000000000000000000 ) ) ;
#44572=ADVANCED_FACE ( 'NONE', ( #21051, #1848 ), #5036, .T. ) ;
#44685=ORIENTED_EDGE ( 'NONE', *, *, #31098, .T. ) ;
#44690=SURFACE_SIDE_STYLE ('',( #51812 ) ) ;
#44699=FACE_OUTER_BOUND ( 'NONE', #33284, .T. ) ;
#44777=VECTOR ( 'NONE', #15901, 1000.000000000000227 ) ;
#44835=DIRECTION ( 'NONE',  ( 0.000000000000000000, 1.000000000000000000, 0.000000000000000000 ) ) ;
#44995=ORIENTED_EDGE ( 'NONE', *, *, #48018, .T. ) ;
#45146=EDGE_CURVE ( 'NONE', #2933, #27449, #11931, .T. ) ;
#45388=EDGE_CURVE ( 'NONE', #42659, #3183, #43861, .T. ) ;
#45485=DIRECTION ( 'NONE',  ( 0.000000000000000000, 1.156482317317871232E-16, 1.000000000000000000 ) ) ;
#45633=EDGE_CURVE ( 'NONE', #46727, #9644, #15128, .T. ) ;
#45748=DIRECTION ( 'NONE',  ( 1.000000000000000000, 0.000000000000000000, 0.000000000000000000 ) ) ;
#45758=ORIENTED_EDGE ( 'NONE', *, *, #41069, .F. ) ;
#45920=DIRECTION ( 'NONE',  ( 0.000000000000000000, 0.000000000000000000, -1.000000000000000000 ) ) ;
#45961=CARTESIAN_POINT ( 'NONE',  ( 0.000000000000000000, -63.50000000000000000, 0.000000000000000000 ) ) ;
#46207=CARTESIAN_POINT ( 'NONE',  ( -365.0160704661291788, -113.5000000000000000, -40.00000000000001421 ) ) ;
#46456=LINE ( 'NONE', #46207, #289 ) ;
#46534=( NAMED_UNIT ( * ) SI_UNIT ( $, .STERADIAN. ) SOLID_ANGLE_UNIT ( ) );
#46638=EDGE_LOOP ( 'NONE', ( #19337, #14894 ) ) ;
#46723=DIRECTION ( 'NONE',  ( 0.000000000000000000, 0.000000000000000000, -1.000000000000000000 ) ) ;
#46727=VERTEX_POINT ( 'NONE', #15615 ) ;
#46978=LINE ( 'NONE', #26980, #19073 ) ;
#46986=DIRECTION ( 'NONE',  ( 0.000000000000000000, 0.000000000000000000, 1.000000000000000000 ) ) ;
#47098=DIRECTION ( 'NONE',  ( 0.000000000000000000, 1.000000000000000000, 0.000000000000000000 ) ) ;
#47209=EDGE_CURVE ( 'NONE', #47963, #27143, #33643, .T. ) ;
#47280=DIRECTION ( 'NONE',  ( 1.000000000000000000, -0.000000000000000000, -0.000000000000000000 ) ) ;
#47351=EDGE_LOOP ( 'NONE', ( #16620, #20551 ) ) ;
#47622=PLANE ( 'NONE',  #17119 ) ;
#47647=DIRECTION ( 'NONE',  ( 0.000000000000000000, -0.8660254037844354880, -0.5000000000000054401 ) ) ;
#47677=CARTESIAN_POINT ( 'NONE',  ( 0.000000000000000000, -63.50000000000000000, -20.00000000000000000 ) ) ;
#47729=PLANE ( 'NONE',  #8192 ) ;
#47851=ADVANCED_FACE ( 'NONE', ( #8755 ), #36885, .F. ) ;
#47925=CARTESIAN_POINT ( 'NONE',  ( -260.0000000000000000, -113.5000000000000000, 39.99999999999998579 ) ) ;
#47963=VERTEX_POINT ( 'NONE', #4303 ) ;
#48016=DIRECTION ( 'NONE',  ( -0.000000000000000000, 0.000000000000000000, -1.000000000000000000 ) ) ;
#48018=EDGE_CURVE ( 'NONE', #12556, #34369, #25067, .T. ) ;
#48315=FACE_OUTER_BOUND ( 'NONE', #22527, .T. ) ;
#48443=ADVANCED_FACE ( 'NONE', ( #42054 ), #50730, .F. ) ;
#48460=LINE ( 'NONE', #12437, #24909 ) ;
#48561=LINE ( 'NONE', #28555, #16913 ) ;
#48635=LINE ( 'NONE', #36517, #19930 ) ;
#48870=EDGE_CURVE ( 'NONE', #13263, #11286, #39006, .T. ) ;
#48891=DIRECTION ( 'NONE',  ( 1.000000000000000000, -0.000000000000000000, -0.000000000000000000 ) ) ;
#49325=LINE ( 'NONE', #20674, #31587 ) ;
#49347=FACE_OUTER_BOUND ( 'NONE', #139, .T. ) ;
#49425=VERTEX_POINT ( 'NONE', #24228 ) ;
#49512=CARTESIAN_POINT ( 'NONE',  ( -260.0000000000000000, -93.50000000000001421, -51.54700538379269403 ) ) ;
#49529=EDGE_CURVE ( 'NONE', #27596, #11286, #25268, .T. ) ;
#49543=PLANE ( 'NONE',  #34676 ) ;
#49584=DIRECTION ( 'NONE',  ( -0.000000000000000000, 1.000000000000000000, -1.541976423090494894E-16 ) ) ;
#49853=PLANE ( 'NONE',  #20927 ) ;
#49981=ORIENTED_EDGE ( 'NONE', *, *, #22092, .T. ) ;
#50053=VECTOR ( 'NONE', #50588, 1000.000000000000000 ) ;
#50123=ORIENTED_EDGE ( 'NONE', *, *, #24688, .T. ) ;
#50185=ORIENTED_EDGE ( 'NONE', *, *, #31239, .T. ) ;
#50272=ORIENTED_EDGE ( 'NONE', *, *, #22869, .F. ) ;
#50342=ADVANCED_FACE ( 'NONE', ( #23579 ), #4143, .F. ) ;
#50358=EDGE_CURVE ( 'NONE', #39530, #22314, #49325, .T. ) ;
#50429=EDGE_CURVE ( 'NONE', #2064, #33404, #32410, .T. ) ;
#50588=DIRECTION ( 'NONE',  ( 0.000000000000000000, 1.000000000000000000, -0.000000000000000000 ) ) ;
#50646=CARTESIAN_POINT ( 'NONE',  ( -280.0000000000000000, -123.5000000000000284, -20.00000000000001066 ) ) ;
#50730=CYLINDRICAL_SURFACE ( 'NONE', #39939, 20.00000000000001776 ) ;
#50875=EDGE_CURVE ( 'NONE', #22314, #27143, #5900, .T. ) ;
#50894=LINE ( 'NONE', #43245, #17415 ) ;
#51073=ADVANCED_FACE ( 'NONE', ( #44699 ), #18344, .F. ) ;
#51112=DIRECTION ( 'NONE',  ( -0.000000000000000000, -1.000000000000000000, -0.000000000000000000 ) ) ;
#51199=ORIENTED_EDGE ( 'NONE', *, *, #39100, .F. ) ;
#51225=CIRCLE ( 'NONE', #28501, 16.00000000000000000 ) ;
#51252=EDGE_CURVE ( 'NONE', #10174, #21356, #46978, .T. ) ;
#51280=ORIENTED_EDGE ( 'NONE', *, *, #14260, .T. ) ;
#51540=FILL_AREA_STYLE ('',( #35753 ) ) ;
#51745=ORIENTED_EDGE ( 'NONE', *, *, #39100, .T. ) ;
#51758=EDGE_LOOP ( 'NONE', ( #12988, #9646, #14793, #15518, #50123, #23358 ) ) ;
#51812=SURFACE_STYLE_FILL_AREA ( #51540 ) ;
#51856=AXIS2_PLACEMENT_3D ( 'NONE', #6120, #10559, #14257 ) ;
ENDSEC;
END-ISO-10303-21;
